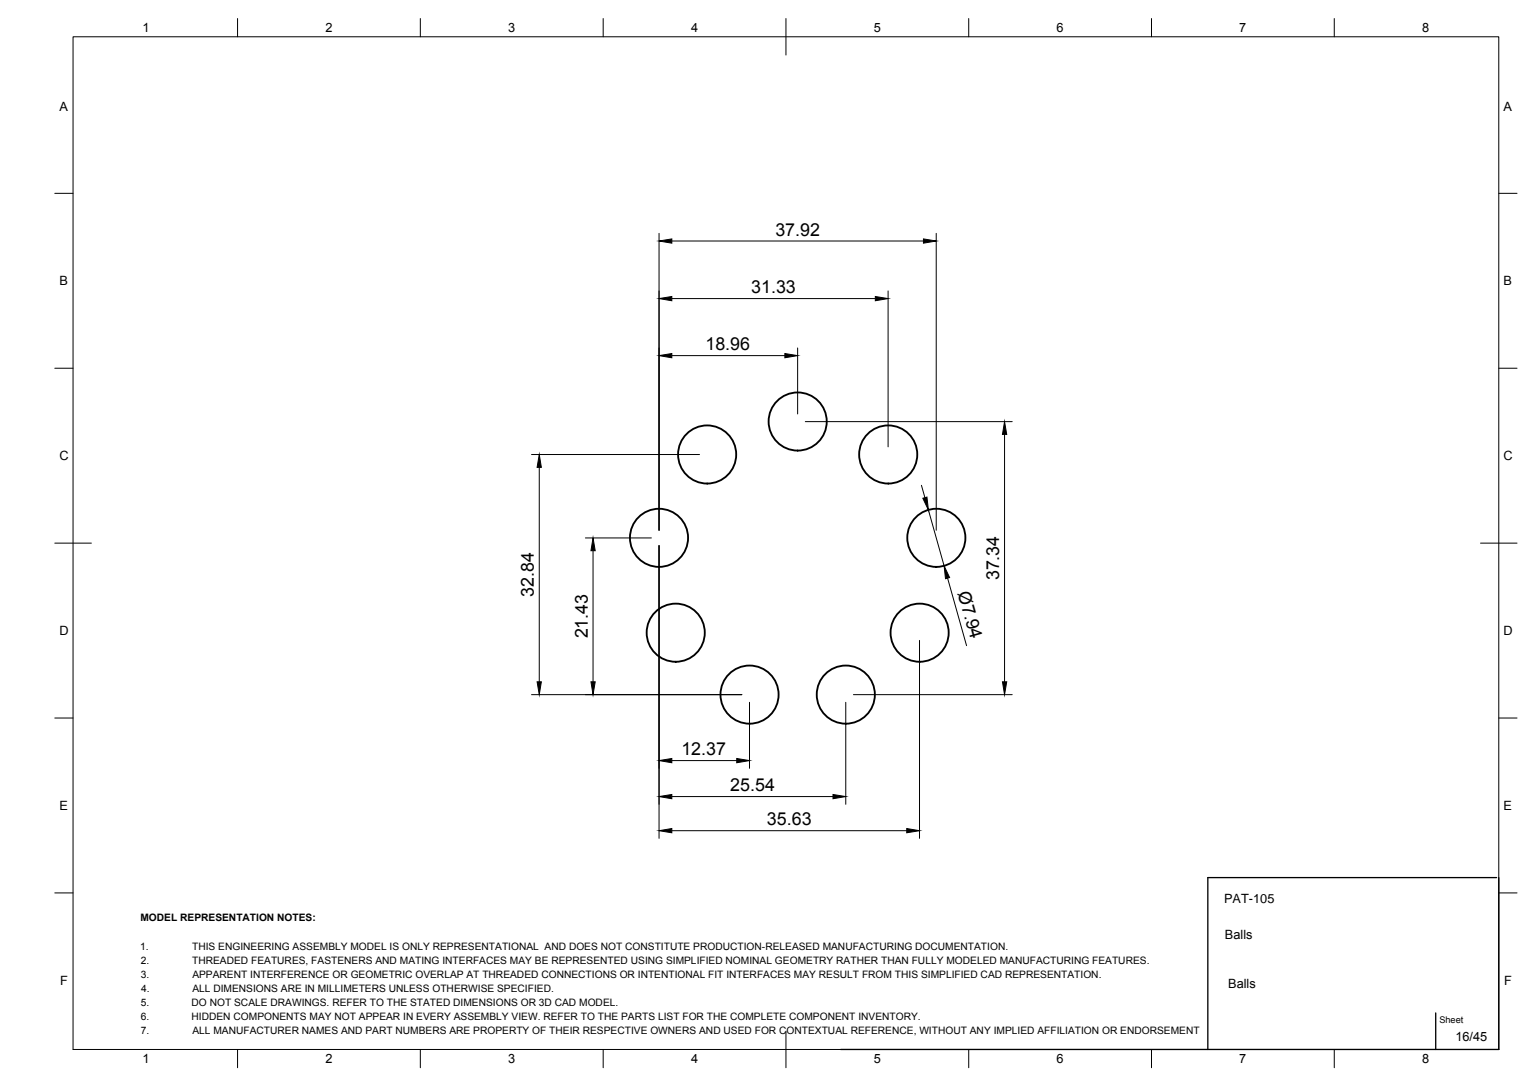
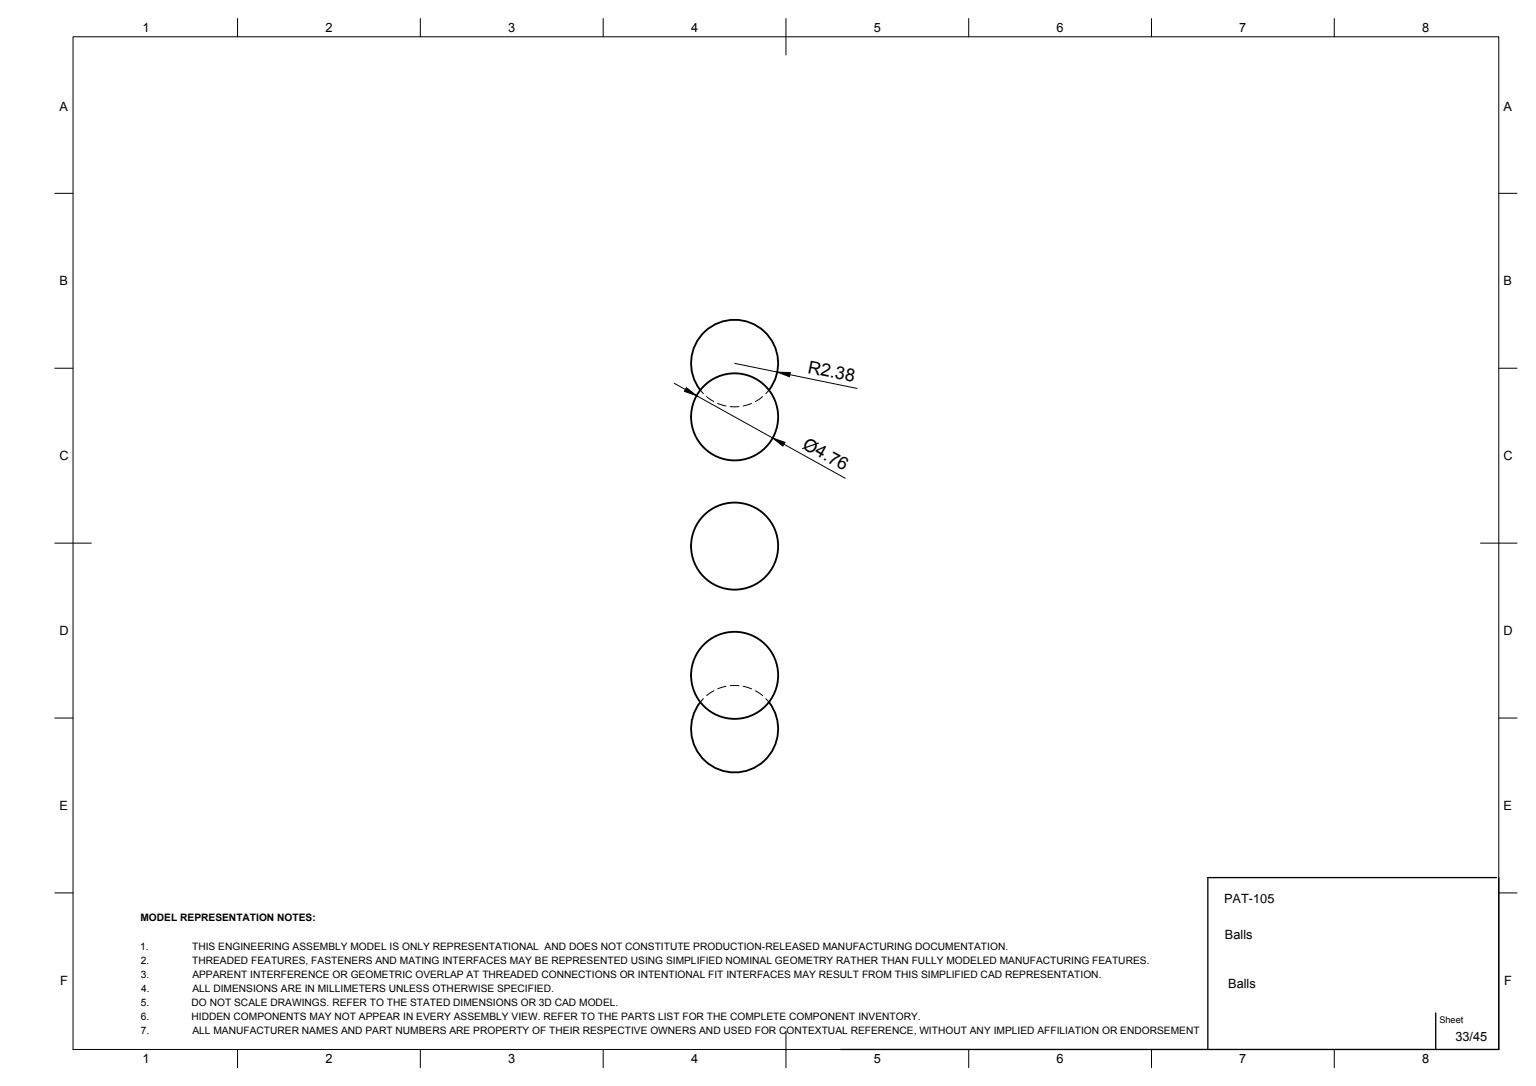
ISO-10303-21;
HEADER;
/* Generated by software containing ST-Developer
 * from STEP Tools, Inc. (www.steptools.com) 
 */

FILE_DESCRIPTION(
/* description */ ('Torque wrench calibration arm'),
/* implementation_level */ '2;1');

FILE_NAME(
/* name */ 'Balls.step',
/* time_stamp */ '2026-10-28T03:24:52-07:00',
/* author */ (''),
/* organization */ (''),
/* preprocessor_version */ 'ST-DEVELOPER v20.2',
/* originating_system */ 'Autodesk Translation Framework v15.17.0.0',
/* authorisation */ '');

FILE_SCHEMA (('AUTOMOTIVE_DESIGN { 1 0 10303 214 3 1 1 }'));
ENDSEC;

DATA;
#10=MECHANICAL_DESIGN_GEOMETRIC_PRESENTATION_REPRESENTATION('',(#435,#436,#437,#438,#439,#440,#441,#442,#443),#12783);
#293=SPHERICAL_SURFACE('',#7199,0.3969);
#294=SPHERICAL_SURFACE('',#7201,0.3969);
#295=SPHERICAL_SURFACE('',#7203,0.3969);
#296=SPHERICAL_SURFACE('',#7205,0.3969);
#297=SPHERICAL_SURFACE('',#7207,0.3969);
#298=SPHERICAL_SURFACE('',#7209,0.3969);
#299=SPHERICAL_SURFACE('',#7211,0.3969);
#300=SPHERICAL_SURFACE('',#7213,0.3969);
#301=SPHERICAL_SURFACE('',#7215,0.3969);
#361=SHAPE_REPRESENTATION_RELATIONSHIP('SRR','None',#12943,#398);
#398=ADVANCED_BREP_SHAPE_REPRESENTATION('',(#489,#490,#491,#492,#493,#494,
#495,#496,#497),#12752);
#435=STYLED_ITEM('',(#13212),#489);
#436=STYLED_ITEM('',(#13212),#490);
#437=STYLED_ITEM('',(#13212),#491);
#438=STYLED_ITEM('',(#13212),#492);
#439=STYLED_ITEM('',(#13212),#493);
#440=STYLED_ITEM('',(#13212),#494);
#441=STYLED_ITEM('',(#13212),#495);
#442=STYLED_ITEM('',(#13212),#496);
#443=STYLED_ITEM('',(#13212),#497);
#489=MANIFOLD_SOLID_BREP('Body1',#6504);
#490=MANIFOLD_SOLID_BREP('Body2',#6505);
#491=MANIFOLD_SOLID_BREP('Body3',#6506);
#492=MANIFOLD_SOLID_BREP('Body4',#6507);
#493=MANIFOLD_SOLID_BREP('Body5',#6508);
#494=MANIFOLD_SOLID_BREP('Body6',#6509);
#495=MANIFOLD_SOLID_BREP('Body7',#6510);
#496=MANIFOLD_SOLID_BREP('Body8',#6511);
#497=MANIFOLD_SOLID_BREP('Body9',#6512);
#991=FACE_OUTER_BOUND('',#1442,.T.);
#992=FACE_OUTER_BOUND('',#1443,.T.);
#993=FACE_OUTER_BOUND('',#1444,.T.);
#994=FACE_OUTER_BOUND('',#1445,.T.);
#995=FACE_OUTER_BOUND('',#1446,.T.);
#996=FACE_OUTER_BOUND('',#1447,.T.);
#997=FACE_OUTER_BOUND('',#1448,.T.);
#998=FACE_OUTER_BOUND('',#1449,.T.);
#999=FACE_OUTER_BOUND('',#1450,.T.);
#1442=EDGE_LOOP('',(#4859,#4860));
#1443=EDGE_LOOP('',(#4861,#4862));
#1444=EDGE_LOOP('',(#4863,#4864));
#1445=EDGE_LOOP('',(#4865,#4866));
#1446=EDGE_LOOP('',(#4867,#4868));
#1447=EDGE_LOOP('',(#4869,#4870));
#1448=EDGE_LOOP('',(#4871,#4872));
#1449=EDGE_LOOP('',(#4873,#4874));
#1450=EDGE_LOOP('',(#4875,#4876));
#2726=CIRCLE('',#7200,0.3969);
#2727=CIRCLE('',#7202,0.3969);
#2728=CIRCLE('',#7204,0.3969);
#2729=CIRCLE('',#7206,0.3969);
#2730=CIRCLE('',#7208,0.3969);
#2731=CIRCLE('',#7210,0.3969);
#2732=CIRCLE('',#7212,0.3969);
#2733=CIRCLE('',#7214,0.3969);
#2734=CIRCLE('',#7216,0.3969);
#3139=VERTEX_POINT('',#10477);
#3140=VERTEX_POINT('',#10478);
#3141=VERTEX_POINT('',#10481);
#3142=VERTEX_POINT('',#10482);
#3143=VERTEX_POINT('',#10485);
#3144=VERTEX_POINT('',#10486);
#3145=VERTEX_POINT('',#10489);
#3146=VERTEX_POINT('',#10490);
#3147=VERTEX_POINT('',#10493);
#3148=VERTEX_POINT('',#10494);
#3149=VERTEX_POINT('',#10497);
#3150=VERTEX_POINT('',#10498);
#3151=VERTEX_POINT('',#10501);
#3152=VERTEX_POINT('',#10502);
#3153=VERTEX_POINT('',#10505);
#3154=VERTEX_POINT('',#10506);
#3155=VERTEX_POINT('',#10509);
#3156=VERTEX_POINT('',#10510);
#3787=EDGE_CURVE('',#3139,#3140,#2726,.T.);
#3788=EDGE_CURVE('',#3141,#3142,#2727,.T.);
#3789=EDGE_CURVE('',#3143,#3144,#2728,.T.);
#3790=EDGE_CURVE('',#3145,#3146,#2729,.T.);
#3791=EDGE_CURVE('',#3147,#3148,#2730,.T.);
#3792=EDGE_CURVE('',#3149,#3150,#2731,.T.);
#3793=EDGE_CURVE('',#3151,#3152,#2732,.T.);
#3794=EDGE_CURVE('',#3153,#3154,#2733,.T.);
#3795=EDGE_CURVE('',#3155,#3156,#2734,.T.);
#4859=ORIENTED_EDGE('',*,*,#3787,.T.);
#4860=ORIENTED_EDGE('',*,*,#3787,.F.);
#4861=ORIENTED_EDGE('',*,*,#3788,.T.);
#4862=ORIENTED_EDGE('',*,*,#3788,.F.);
#4863=ORIENTED_EDGE('',*,*,#3789,.T.);
#4864=ORIENTED_EDGE('',*,*,#3789,.F.);
#4865=ORIENTED_EDGE('',*,*,#3790,.T.);
#4866=ORIENTED_EDGE('',*,*,#3790,.F.);
#4867=ORIENTED_EDGE('',*,*,#3791,.T.);
#4868=ORIENTED_EDGE('',*,*,#3791,.F.);
#4869=ORIENTED_EDGE('',*,*,#3792,.T.);
#4870=ORIENTED_EDGE('',*,*,#3792,.F.);
#4871=ORIENTED_EDGE('',*,*,#3793,.T.);
#4872=ORIENTED_EDGE('',*,*,#3793,.F.);
#4873=ORIENTED_EDGE('',*,*,#3794,.T.);
#4874=ORIENTED_EDGE('',*,*,#3794,.F.);
#4875=ORIENTED_EDGE('',*,*,#3795,.T.);
#4876=ORIENTED_EDGE('',*,*,#3795,.F.);
#6216=ADVANCED_FACE('',(#991),#293,.T.);
#6217=ADVANCED_FACE('',(#992),#294,.T.);
#6218=ADVANCED_FACE('',(#993),#295,.T.);
#6219=ADVANCED_FACE('',(#994),#296,.T.);
#6220=ADVANCED_FACE('',(#995),#297,.T.);
#6221=ADVANCED_FACE('',(#996),#298,.T.);
#6222=ADVANCED_FACE('',(#997),#299,.T.);
#6223=ADVANCED_FACE('',(#998),#300,.T.);
#6224=ADVANCED_FACE('',(#999),#301,.T.);
#6504=CLOSED_SHELL('',(#6216));
#6505=CLOSED_SHELL('',(#6217));
#6506=CLOSED_SHELL('',(#6218));
#6507=CLOSED_SHELL('',(#6219));
#6508=CLOSED_SHELL('',(#6220));
#6509=CLOSED_SHELL('',(#6221));
#6510=CLOSED_SHELL('',(#6222));
#6511=CLOSED_SHELL('',(#6223));
#6512=CLOSED_SHELL('',(#6224));
#7198=AXIS2_PLACEMENT_3D('',#10475,#8430,#8431);
#7199=AXIS2_PLACEMENT_3D('',#10476,#8432,#8433);
#7200=AXIS2_PLACEMENT_3D('',#10479,#8434,#8435);
#7201=AXIS2_PLACEMENT_3D('',#10480,#8436,#8437);
#7202=AXIS2_PLACEMENT_3D('',#10483,#8438,#8439);
#7203=AXIS2_PLACEMENT_3D('',#10484,#8440,#8441);
#7204=AXIS2_PLACEMENT_3D('',#10487,#8442,#8443);
#7205=AXIS2_PLACEMENT_3D('',#10488,#8444,#8445);
#7206=AXIS2_PLACEMENT_3D('',#10491,#8446,#8447);
#7207=AXIS2_PLACEMENT_3D('',#10492,#8448,#8449);
#7208=AXIS2_PLACEMENT_3D('',#10495,#8450,#8451);
#7209=AXIS2_PLACEMENT_3D('',#10496,#8452,#8453);
#7210=AXIS2_PLACEMENT_3D('',#10499,#8454,#8455);
#7211=AXIS2_PLACEMENT_3D('',#10500,#8456,#8457);
#7212=AXIS2_PLACEMENT_3D('',#10503,#8458,#8459);
#7213=AXIS2_PLACEMENT_3D('',#10504,#8460,#8461);
#7214=AXIS2_PLACEMENT_3D('',#10507,#8462,#8463);
#7215=AXIS2_PLACEMENT_3D('',#10508,#8464,#8465);
#7216=AXIS2_PLACEMENT_3D('',#10511,#8466,#8467);
#8430=DIRECTION('axis',(0.,0.,1.));
#8431=DIRECTION('refdir',(1.,0.,0.));
#8432=DIRECTION('center_axis',(0.,0.,1.));
#8433=DIRECTION('ref_axis',(1.,0.,0.));
#8434=DIRECTION('center_axis',(1.22464679914735E-16,-1.,0.));
#8435=DIRECTION('ref_axis',(-1.,-1.22464679914735E-16,0.));
#8436=DIRECTION('center_axis',(0.642787609686539,0.,0.766044443118978));
#8437=DIRECTION('ref_axis',(0.766044443118978,0.,-0.642787609686539));
#8438=DIRECTION('center_axis',(9.38133875270273E-17,-1.,-7.87187788734199E-17));
#8439=DIRECTION('ref_axis',(-0.766044443118978,-1.22464679914735E-16,0.642787609686539));
#8440=DIRECTION('center_axis',(0.984807753012208,0.,0.173648177666931));
#8441=DIRECTION('ref_axis',(0.17364817766693,0.,-0.984807753012208));
#8442=DIRECTION('center_axis',(2.12657684957577E-17,-1.,-1.2060416625019E-16));
#8443=DIRECTION('ref_axis',(-0.17364817766693,-1.22464679914735E-16,0.984807753012208));
#8444=DIRECTION('center_axis',(0.866025403784439,0.,-0.5));
#8445=DIRECTION('ref_axis',(-0.5,0.,-0.866025403784439));
#8446=DIRECTION('center_axis',(-6.12323399573676E-17,-1.,-1.06057523872491E-16));
#8447=DIRECTION('ref_axis',(0.5,-1.22464679914735E-16,0.866025403784439));
#8448=DIRECTION('center_axis',(0.342020143325669,0.,-0.939692620785908));
#8449=DIRECTION('ref_axis',(-0.939692620785908,0.,-0.342020143325669));
#8450=DIRECTION('center_axis',(-1.15079156022785E-16,-1.,-4.18853873767699E-17));
#8451=DIRECTION('ref_axis',(0.939692620785908,-1.22464679914735E-16,0.342020143325669));
#8452=DIRECTION('center_axis',(-0.342020143325669,0.,-0.939692620785908));
#8453=DIRECTION('ref_axis',(-0.939692620785909,0.,0.342020143325669));
#8454=DIRECTION('center_axis',(-1.15079156022785E-16,-1.,4.18853873767699E-17));
#8455=DIRECTION('ref_axis',(0.939692620785908,-1.22464679914735E-16,-0.342020143325669));
#8456=DIRECTION('center_axis',(-0.866025403784438,0.,-0.5));
#8457=DIRECTION('ref_axis',(-0.5,0.,0.866025403784438));
#8458=DIRECTION('center_axis',(-6.12323399573677E-17,-1.,1.06057523872491E-16));
#8459=DIRECTION('ref_axis',(0.5,-1.22464679914735E-16,-0.866025403784438));
#8460=DIRECTION('center_axis',(-0.984807753012208,0.,0.17364817766693));
#8461=DIRECTION('ref_axis',(0.17364817766693,0.,0.984807753012208));
#8462=DIRECTION('center_axis',(2.12657684957577E-17,-1.,1.2060416625019E-16));
#8463=DIRECTION('ref_axis',(-0.17364817766693,-1.22464679914735E-16,-0.984807753012208));
#8464=DIRECTION('center_axis',(-0.64278760968654,0.,0.766044443118978));
#8465=DIRECTION('ref_axis',(0.766044443118978,0.,0.64278760968654));
#8466=DIRECTION('center_axis',(9.38133875270273E-17,-1.,7.87187788734199E-17));
#8467=DIRECTION('ref_axis',(-0.766044443118978,-1.22464679914735E-16,-0.64278760968654));
#10475=CARTESIAN_POINT('',(0.,0.,0.));
#10476=CARTESIAN_POINT('Origin',(1.925,0.,0.));
#10477=CARTESIAN_POINT('',(1.925,-2.97627328869245E-33,0.3969));
#10478=CARTESIAN_POINT('',(1.925,-2.97627328869245E-33,-0.3969));
#10479=CARTESIAN_POINT('Origin',(1.925,0.,0.));
#10480=CARTESIAN_POINT('Origin',(1.47463555300403,0.,-1.23736614864659));
#10481=CARTESIAN_POINT('',(1.72975795528862,-2.97627328869245E-33,-0.933323109172666));
#10482=CARTESIAN_POINT('',(1.21951315071945,-2.97627328869245E-33,-1.54140918812051));
#10483=CARTESIAN_POINT('Origin',(1.47463555300403,0.,-1.23736614864659));
#10484=CARTESIAN_POINT('Origin',(0.334272742008841,0.,-1.8957549245485));
#10485=CARTESIAN_POINT('',(0.725142939179386,1.05214622327121E-34,-1.8268339628325));
#10486=CARTESIAN_POINT('',(-0.0565974551617042,-6.05776119971203E-33,-1.96467588626451));
#10487=CARTESIAN_POINT('Origin',(0.334272742008841,0.,-1.8957549245485));
#10488=CARTESIAN_POINT('Origin',(-0.9625,0.,-1.66709890228504));
#10489=CARTESIAN_POINT('',(-0.618774517237956,-2.97627328869245E-33,-1.86554890228504));
#10490=CARTESIAN_POINT('',(-1.30622548276204,-2.97627328869245E-33,-1.46864890228504));
#10491=CARTESIAN_POINT('Origin',(-0.9625,0.,-1.66709890228504));
#10492=CARTESIAN_POINT('Origin',(-1.80890829501287,0.,-0.658388775901913));
#10493=CARTESIAN_POINT('',(-1.67316050012692,1.05214622327121E-34,-1.03135277709184));
#10494=CARTESIAN_POINT('',(-1.94465608989883,-6.05776119971203E-33,-0.285424774711986));
#10495=CARTESIAN_POINT('Origin',(-1.80890829501287,0.,-0.658388775901913));
#10496=CARTESIAN_POINT('Origin',(-1.80890829501287,0.,0.658388775901912));
#10497=CARTESIAN_POINT('',(-1.94465608989883,-9.13924911073161E-33,0.285424774711985));
#10498=CARTESIAN_POINT('',(-1.67316050012692,3.1867025333467E-33,1.03135277709184));
#10499=CARTESIAN_POINT('Origin',(-1.80890829501287,0.,0.658388775901912));
#10500=CARTESIAN_POINT('Origin',(-0.962500000000001,0.,1.66709890228504));
#10501=CARTESIAN_POINT('',(-1.30622548276204,-2.97627328869245E-33,1.46864890228504));
#10502=CARTESIAN_POINT('',(-0.618774517237957,-2.97627328869245E-33,1.86554890228504));
#10503=CARTESIAN_POINT('Origin',(-0.962500000000001,0.,1.66709890228504));
#10504=CARTESIAN_POINT('Origin',(0.33427274200884,0.,1.8957549245485));
#10505=CARTESIAN_POINT('',(-0.0565974551617051,-2.97627328869245E-33,1.96467588626451));
#10506=CARTESIAN_POINT('',(0.725142939179386,-2.97627328869245E-33,1.8268339628325));
#10507=CARTESIAN_POINT('Origin',(0.33427274200884,0.,1.8957549245485));
#10508=CARTESIAN_POINT('Origin',(1.47463555300403,0.,1.23736614864659));
#10509=CARTESIAN_POINT('',(1.21951315071944,-6.05776119971203E-33,1.54140918812051));
#10510=CARTESIAN_POINT('',(1.72975795528862,1.05214622327122E-34,0.933323109172667));
#10511=CARTESIAN_POINT('Origin',(1.47463555300403,0.,1.23736614864659));
#12708=UNCERTAINTY_MEASURE_WITH_UNIT(LENGTH_MEASURE(0.001),#12784,
'DISTANCE_ACCURACY_VALUE',
'Maximum model space distance between geometric entities at asserted c
onnectivities');
#12739=UNCERTAINTY_MEASURE_WITH_UNIT(LENGTH_MEASURE(0.001),#12784,
'DISTANCE_ACCURACY_VALUE',
'Maximum model space distance between geometric entities at asserted c
onnectivities');
#12752=(
GEOMETRIC_REPRESENTATION_CONTEXT(3)
GLOBAL_UNCERTAINTY_ASSIGNED_CONTEXT((#12708))
GLOBAL_UNIT_ASSIGNED_CONTEXT((#12784,#12786,#12787))
REPRESENTATION_CONTEXT('','3D')
);
#12783=(
GEOMETRIC_REPRESENTATION_CONTEXT(3)
GLOBAL_UNCERTAINTY_ASSIGNED_CONTEXT((#12739))
GLOBAL_UNIT_ASSIGNED_CONTEXT((#12784,#12786,#12787))
REPRESENTATION_CONTEXT('','3D')
);
#12784=(
LENGTH_UNIT()
NAMED_UNIT(*)
SI_UNIT(.CENTI.,.METRE.)
);
#12786=(
NAMED_UNIT(*)
PLANE_ANGLE_UNIT()
SI_UNIT($,.RADIAN.)
);
#12787=(
NAMED_UNIT(*)
SI_UNIT($,.STERADIAN.)
SOLID_ANGLE_UNIT()
);
#12800=SHAPE_DEFINITION_REPRESENTATION(#12843,#12943);
#12843=PRODUCT_DEFINITION_SHAPE('',$,#12987);
#12943=SHAPE_REPRESENTATION('',(#7198),#12752);
#12974=PRODUCT_DEFINITION_CONTEXT('part definition',#13105,'design');
#12987=PRODUCT_DEFINITION('Balls','Balls',#13030,#12974);
#13030=PRODUCT_DEFINITION_FORMATION('',$,#13119);
#13105=APPLICATION_CONTEXT(
'Core Data for Automotive Mechanical Design Process');
#13106=PRODUCT_CONTEXT('part definition',#13105,'mechanical');
#13119=PRODUCT('Balls','Balls','Balls',(#13106));
#13206=COLOUR_RGB('Grey',0.48,0.52,0.57);
#13207=FILL_AREA_STYLE_COLOUR('',#13206);
#13208=FILL_AREA_STYLE('',(#13207));
#13209=SURFACE_STYLE_FILL_AREA(#13208);
#13210=SURFACE_SIDE_STYLE('',(#13209));
#13211=SURFACE_STYLE_USAGE(.BOTH.,#13210);
#13212=PRESENTATION_STYLE_ASSIGNMENT((#13211));
ENDSEC;
END-ISO-10303-21;
